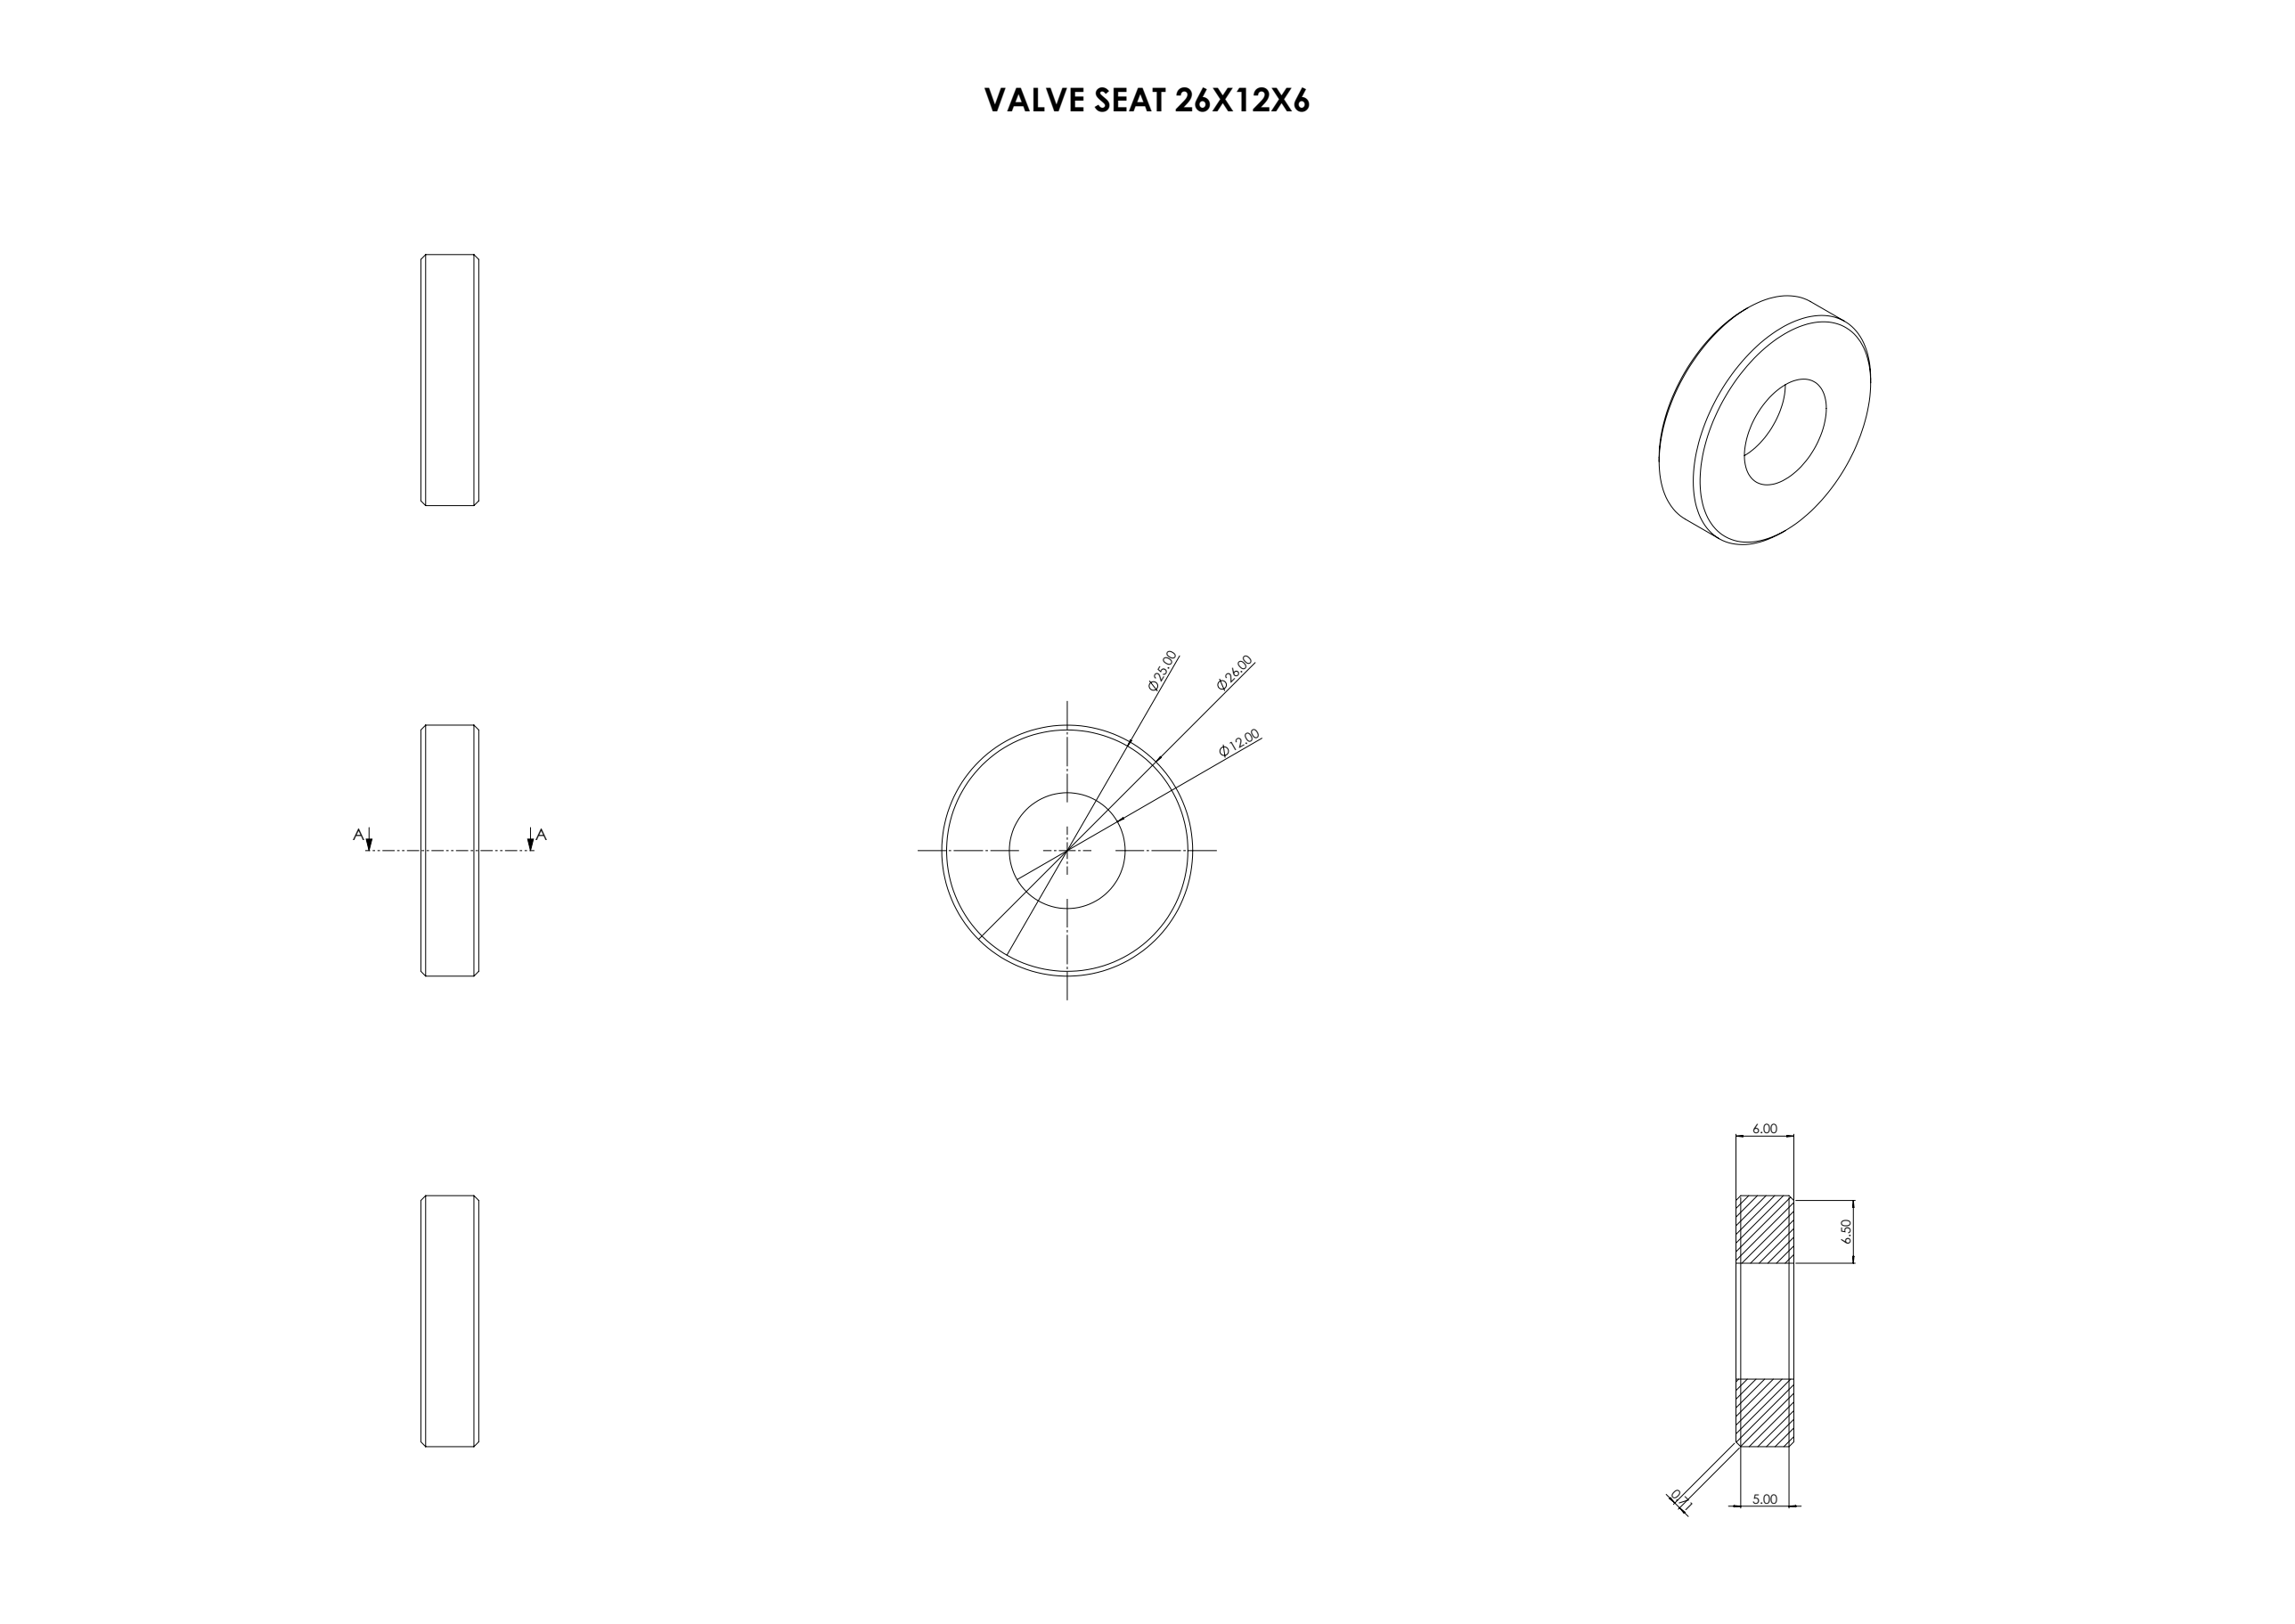
ISO-10303-21;
HEADER;
/* Generated by software containing ST-Developer
 * from STEP Tools, Inc. (www.steptools.com) 
 */

FILE_DESCRIPTION(
/* description */ (''),
/* implementation_level */ '2;1');

FILE_NAME(
/* name */ '13_Valve_Seat_26x12x6.step',
/* time_stamp */ '2026-10-26T06:13:19-07:00',
/* author */ (''),
/* organization */ (''),
/* preprocessor_version */ 'ST-DEVELOPER v20.2',
/* originating_system */ 'Autodesk Translation Framework v15.15.0.0',
/* authorisation */ '');

FILE_SCHEMA (('AUTOMOTIVE_DESIGN { 1 0 10303 214 3 1 1 }','TECHNICAL_DATA_PACKAGING'));
ENDSEC;

DATA;
#10=MECHANICAL_DESIGN_GEOMETRIC_PRESENTATION_REPRESENTATION('',(#311),#56639);
#271=SHAPE_REPRESENTATION_RELATIONSHIP('SRR','None',#56759,#291);
#291=ADVANCED_BREP_SHAPE_REPRESENTATION('',(#331),#56633);
#311=STYLED_ITEM('',(#56908),#331);
#331=MANIFOLD_SOLID_BREP('Body1',#16963);
#545=FACE_BOUND('',#3452,.T.);
#546=FACE_BOUND('',#3457,.T.);
#621=CONICAL_SURFACE('',#18211,12.75,0.785398163397449);
#622=CONICAL_SURFACE('',#18215,12.75,0.78539816339745);
#1126=CIRCLE('',#18207,6.);
#1127=CIRCLE('',#18208,6.);
#1128=CIRCLE('',#18210,12.5);
#1129=CIRCLE('',#18212,13.);
#1130=CIRCLE('',#18214,13.);
#1131=CIRCLE('',#18216,12.5);
#1454=CYLINDRICAL_SURFACE('',#18206,6.);
#1455=CYLINDRICAL_SURFACE('',#18213,13.);
#2346=FACE_OUTER_BOUND('',#3450,.T.);
#2347=FACE_OUTER_BOUND('',#3451,.T.);
#2348=FACE_OUTER_BOUND('',#3453,.T.);
#2349=FACE_OUTER_BOUND('',#3454,.T.);
#2350=FACE_OUTER_BOUND('',#3455,.T.);
#2351=FACE_OUTER_BOUND('',#3456,.T.);
#3450=EDGE_LOOP('',(#13344,#13345,#13346,#13347));
#3451=EDGE_LOOP('',(#13348));
#3452=EDGE_LOOP('',(#13349));
#3453=EDGE_LOOP('',(#13350,#13351,#13352,#13353));
#3454=EDGE_LOOP('',(#13354,#13355,#13356,#13357));
#3455=EDGE_LOOP('',(#13358,#13359,#13360,#13361));
#3456=EDGE_LOOP('',(#13362));
#3457=EDGE_LOOP('',(#13363));
#4421=LINE('',#36438,#5375);
#4422=LINE('',#36446,#5376);
#4423=LINE('',#36450,#5377);
#4424=LINE('',#36454,#5378);
#5375=VECTOR('',#21345,6.);
#5376=VECTOR('',#21356,12.75);
#5377=VECTOR('',#21361,13.);
#5378=VECTOR('',#21366,12.75);
#7521=VERTEX_POINT('',#36435);
#7522=VERTEX_POINT('',#36437);
#7523=VERTEX_POINT('',#36441);
#7524=VERTEX_POINT('',#36444);
#7525=VERTEX_POINT('',#36448);
#7526=VERTEX_POINT('',#36452);
#9579=EDGE_CURVE('',#7521,#7521,#1126,.T.);
#9580=EDGE_CURVE('',#7521,#7522,#4421,.T.);
#9581=EDGE_CURVE('',#7522,#7522,#1127,.T.);
#9582=EDGE_CURVE('',#7523,#7523,#1128,.T.);
#9583=EDGE_CURVE('',#7524,#7524,#1129,.T.);
#9584=EDGE_CURVE('',#7524,#7523,#4422,.T.);
#9585=EDGE_CURVE('',#7525,#7525,#1130,.T.);
#9586=EDGE_CURVE('',#7525,#7524,#4423,.T.);
#9587=EDGE_CURVE('',#7526,#7526,#1131,.T.);
#9588=EDGE_CURVE('',#7526,#7525,#4424,.T.);
#13344=ORIENTED_EDGE('',*,*,#9579,.T.);
#13345=ORIENTED_EDGE('',*,*,#9580,.T.);
#13346=ORIENTED_EDGE('',*,*,#9581,.F.);
#13347=ORIENTED_EDGE('',*,*,#9580,.F.);
#13348=ORIENTED_EDGE('',*,*,#9582,.F.);
#13349=ORIENTED_EDGE('',*,*,#9581,.T.);
#13350=ORIENTED_EDGE('',*,*,#9583,.F.);
#13351=ORIENTED_EDGE('',*,*,#9584,.T.);
#13352=ORIENTED_EDGE('',*,*,#9582,.T.);
#13353=ORIENTED_EDGE('',*,*,#9584,.F.);
#13354=ORIENTED_EDGE('',*,*,#9585,.F.);
#13355=ORIENTED_EDGE('',*,*,#9586,.T.);
#13356=ORIENTED_EDGE('',*,*,#9583,.T.);
#13357=ORIENTED_EDGE('',*,*,#9586,.F.);
#13358=ORIENTED_EDGE('',*,*,#9587,.F.);
#13359=ORIENTED_EDGE('',*,*,#9588,.T.);
#13360=ORIENTED_EDGE('',*,*,#9585,.T.);
#13361=ORIENTED_EDGE('',*,*,#9588,.F.);
#13362=ORIENTED_EDGE('',*,*,#9587,.T.);
#13363=ORIENTED_EDGE('',*,*,#9579,.F.);
#15904=PLANE('',#18209);
#15905=PLANE('',#18217);
#16517=ADVANCED_FACE('',(#2346),#1454,.F.);
#16518=ADVANCED_FACE('',(#2347,#545),#15904,.T.);
#16519=ADVANCED_FACE('',(#2348),#621,.T.);
#16520=ADVANCED_FACE('',(#2349),#1455,.T.);
#16521=ADVANCED_FACE('',(#2350),#622,.T.);
#16522=ADVANCED_FACE('',(#2351,#546),#15905,.T.);
#16963=CLOSED_SHELL('',(#16517,#16518,#16519,#16520,#16521,#16522));
#18205=AXIS2_PLACEMENT_3D('',#36433,#21339,#21340);
#18206=AXIS2_PLACEMENT_3D('',#36434,#21341,#21342);
#18207=AXIS2_PLACEMENT_3D('',#36436,#21343,#21344);
#18208=AXIS2_PLACEMENT_3D('',#36439,#21346,#21347);
#18209=AXIS2_PLACEMENT_3D('',#36440,#21348,#21349);
#18210=AXIS2_PLACEMENT_3D('',#36442,#21350,#21351);
#18211=AXIS2_PLACEMENT_3D('',#36443,#21352,#21353);
#18212=AXIS2_PLACEMENT_3D('',#36445,#21354,#21355);
#18213=AXIS2_PLACEMENT_3D('',#36447,#21357,#21358);
#18214=AXIS2_PLACEMENT_3D('',#36449,#21359,#21360);
#18215=AXIS2_PLACEMENT_3D('',#36451,#21362,#21363);
#18216=AXIS2_PLACEMENT_3D('',#36453,#21364,#21365);
#18217=AXIS2_PLACEMENT_3D('',#36455,#21367,#21368);
#21339=DIRECTION('axis',(0.,0.,1.));
#21340=DIRECTION('refdir',(1.,0.,0.));
#21341=DIRECTION('center_axis',(1.,0.,0.));
#21342=DIRECTION('ref_axis',(0.,1.,0.));
#21343=DIRECTION('center_axis',(1.,0.,0.));
#21344=DIRECTION('ref_axis',(0.,0.,-1.));
#21345=DIRECTION('',(-1.,0.,0.));
#21346=DIRECTION('center_axis',(1.,0.,0.));
#21347=DIRECTION('ref_axis',(0.,0.,-1.));
#21348=DIRECTION('center_axis',(-1.,0.,0.));
#21349=DIRECTION('ref_axis',(0.,0.,1.));
#21350=DIRECTION('center_axis',(1.,0.,0.));
#21351=DIRECTION('ref_axis',(0.,0.,-1.));
#21352=DIRECTION('center_axis',(1.,0.,0.));
#21353=DIRECTION('ref_axis',(0.,1.,0.));
#21354=DIRECTION('center_axis',(1.,0.,0.));
#21355=DIRECTION('ref_axis',(0.,0.,-1.));
#21356=DIRECTION('',(-0.707106781186547,0.707106781186548,8.65956056235494E-17));
#21357=DIRECTION('center_axis',(1.,0.,0.));
#21358=DIRECTION('ref_axis',(0.,1.,0.));
#21359=DIRECTION('center_axis',(1.,0.,0.));
#21360=DIRECTION('ref_axis',(0.,0.,-1.));
#21361=DIRECTION('',(-1.,0.,0.));
#21362=DIRECTION('center_axis',(-1.,0.,0.));
#21363=DIRECTION('ref_axis',(0.,1.,0.));
#21364=DIRECTION('center_axis',(1.,0.,0.));
#21365=DIRECTION('ref_axis',(0.,0.,-1.));
#21366=DIRECTION('',(-0.707106781186547,-0.707106781186548,-8.65956056235494E-17));
#21367=DIRECTION('center_axis',(1.,0.,0.));
#21368=DIRECTION('ref_axis',(0.,0.,-1.));
#36433=CARTESIAN_POINT('',(0.,0.,0.));
#36434=CARTESIAN_POINT('Origin',(3.,0.,0.));
#36435=CARTESIAN_POINT('',(6.,-6.,-7.34788079488412E-16));
#36436=CARTESIAN_POINT('Origin',(6.,0.,0.));
#36437=CARTESIAN_POINT('',(0.,-6.,-7.34788079488412E-16));
#36438=CARTESIAN_POINT('',(3.,-6.,-7.34788079488412E-16));
#36439=CARTESIAN_POINT('Origin',(0.,0.,0.));
#36440=CARTESIAN_POINT('Origin',(0.,12.5,0.));
#36441=CARTESIAN_POINT('',(6.93889390390723E-17,-12.5,-1.53080849893419E-15));
#36442=CARTESIAN_POINT('Origin',(0.,0.,0.));
#36443=CARTESIAN_POINT('Origin',(0.25,0.,0.));
#36444=CARTESIAN_POINT('',(0.500000000000001,-13.,-1.59204083889156E-15));
#36445=CARTESIAN_POINT('Origin',(0.5,0.,0.));
#36446=CARTESIAN_POINT('',(0.25,-12.75,-1.56142466891288E-15));
#36447=CARTESIAN_POINT('Origin',(3.,0.,0.));
#36448=CARTESIAN_POINT('',(5.5,-13.,-1.59204083889156E-15));
#36449=CARTESIAN_POINT('Origin',(5.5,0.,0.));
#36450=CARTESIAN_POINT('',(3.,-13.,-1.59204083889156E-15));
#36451=CARTESIAN_POINT('Origin',(5.75,0.,0.));
#36452=CARTESIAN_POINT('',(6.,-12.5,-1.53080849893419E-15));
#36453=CARTESIAN_POINT('Origin',(6.,0.,0.));
#36454=CARTESIAN_POINT('',(5.75,-12.75,-1.56142466891288E-15));
#36455=CARTESIAN_POINT('Origin',(6.,6.,0.));
#56611=UNCERTAINTY_MEASURE_WITH_UNIT(LENGTH_MEASURE(0.01),#56640,
'DISTANCE_ACCURACY_VALUE',
'Maximum model space distance between geometric entities at asserted c
onnectivities');
#56617=UNCERTAINTY_MEASURE_WITH_UNIT(LENGTH_MEASURE(0.01),#56640,
'DISTANCE_ACCURACY_VALUE',
'Maximum model space distance between geometric entities at asserted c
onnectivities');
#56633=(
GEOMETRIC_REPRESENTATION_CONTEXT(3)
GLOBAL_UNCERTAINTY_ASSIGNED_CONTEXT((#56611))
GLOBAL_UNIT_ASSIGNED_CONTEXT((#56640,#56642,#56643))
REPRESENTATION_CONTEXT('','3D')
);
#56639=(
GEOMETRIC_REPRESENTATION_CONTEXT(3)
GLOBAL_UNCERTAINTY_ASSIGNED_CONTEXT((#56617))
GLOBAL_UNIT_ASSIGNED_CONTEXT((#56640,#56642,#56643))
REPRESENTATION_CONTEXT('','3D')
);
#56640=(
LENGTH_UNIT()
NAMED_UNIT(*)
SI_UNIT(.MILLI.,.METRE.)
);
#56642=(
NAMED_UNIT(*)
PLANE_ANGLE_UNIT()
SI_UNIT($,.RADIAN.)
);
#56643=(
NAMED_UNIT(*)
SI_UNIT($,.STERADIAN.)
SOLID_ANGLE_UNIT()
);
#56659=SHAPE_DEFINITION_REPRESENTATION(#56680,#56759);
#56680=PRODUCT_DEFINITION_SHAPE('',$,#56781);
#56759=SHAPE_REPRESENTATION('',(#18205),#56633);
#56765=PRODUCT_DEFINITION_CONTEXT('part definition',#56830,'design');
#56781=PRODUCT_DEFINITION('2026-10-26-00-02-50-406',
'13_Valve_Seat_26x12x6',#56802,#56765);
#56802=PRODUCT_DEFINITION_FORMATION('',$,#56847);
#56830=APPLICATION_CONTEXT(
'Core Data for Automotive Mechanical Design Process');
#56831=PRODUCT_CONTEXT('part definition',#56830,'mechanical');
#56847=PRODUCT('2026-10-26-00-02-50-406','13_Valve_Seat_26x12x6',$,(#56831));
#56902=COLOUR_RGB('Sky Blue',0.24,0.69,0.87);
#56903=FILL_AREA_STYLE_COLOUR('',#56902);
#56904=FILL_AREA_STYLE('',(#56903));
#56905=SURFACE_STYLE_FILL_AREA(#56904);
#56906=SURFACE_SIDE_STYLE('',(#56905));
#56907=SURFACE_STYLE_USAGE(.BOTH.,#56906);
#56908=PRESENTATION_STYLE_ASSIGNMENT((#56907));
ENDSEC;
END-ISO-10303-21;
